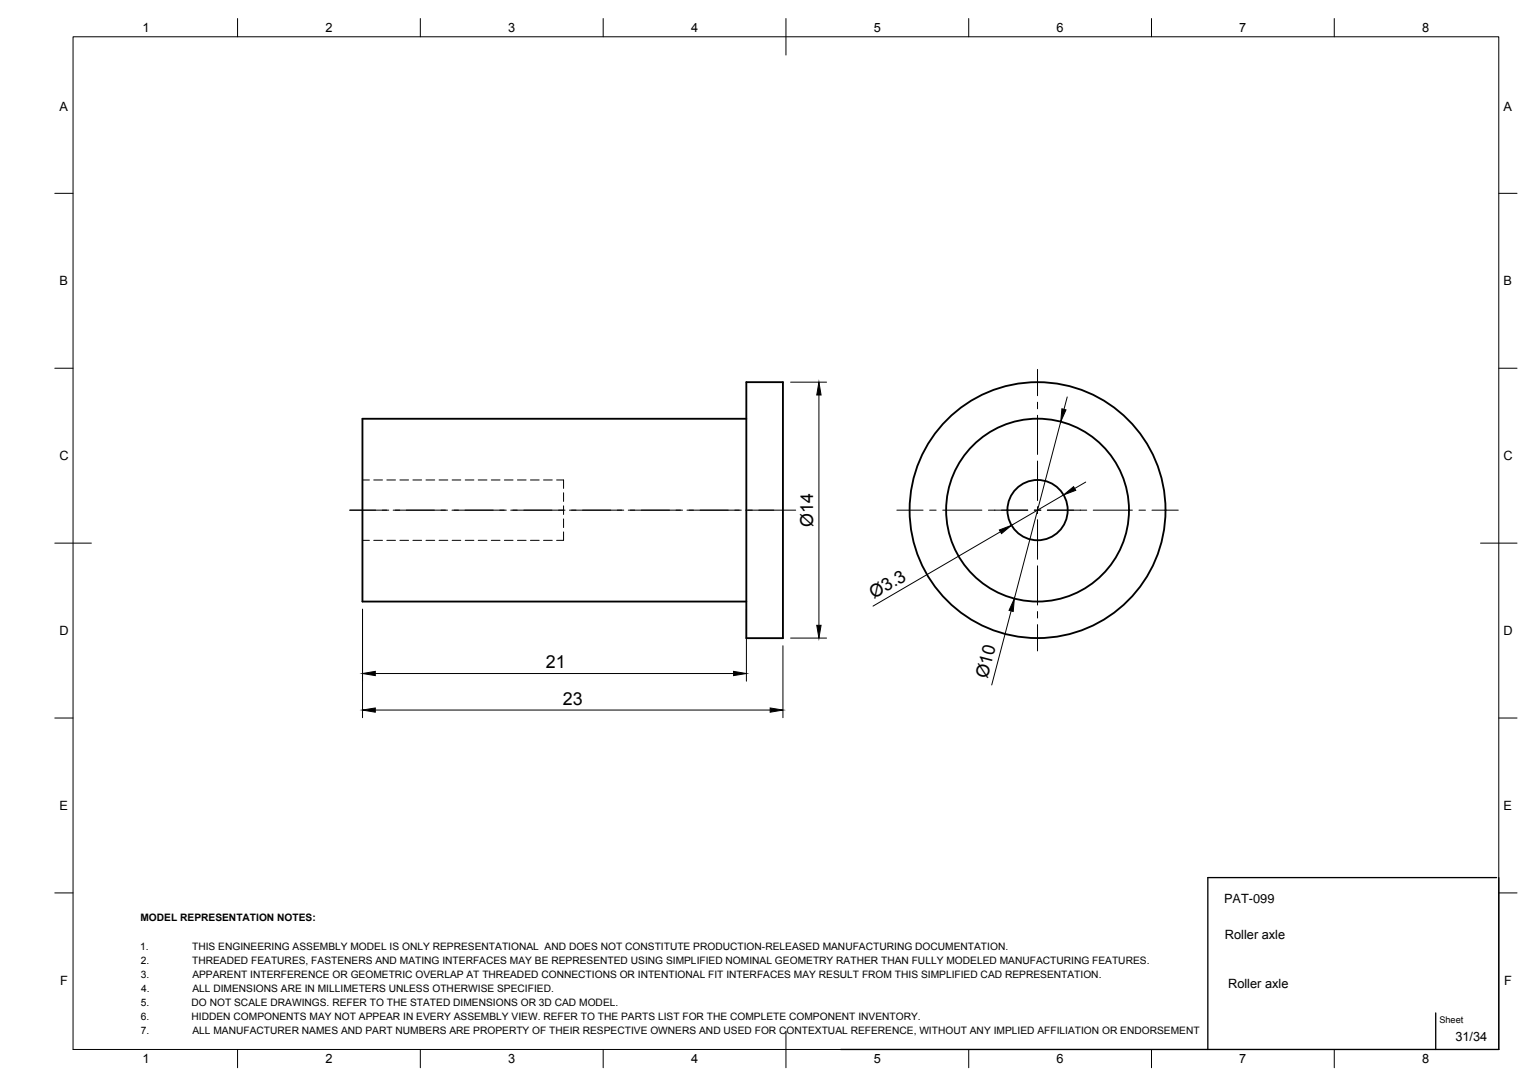
ISO-10303-21;
HEADER;
/* Generated by software containing ST-Developer
 * from STEP Tools, Inc. (www.steptools.com) 
 */

FILE_DESCRIPTION(
/* description */ ('PAT-099'),
/* implementation_level */ '2;1');

FILE_NAME(
/* name */ 'Roller axle.step',
/* time_stamp */ '2026-10-29T17:25:42-07:00',
/* author */ (''),
/* organization */ (''),
/* preprocessor_version */ 'ST-DEVELOPER v20.2',
/* originating_system */ 'Autodesk Translation Framework v15.17.0.0',
/* authorisation */ '');

FILE_SCHEMA (('AUTOMOTIVE_DESIGN { 1 0 10303 214 3 1 1 }'));
ENDSEC;

DATA;
#10=MECHANICAL_DESIGN_GEOMETRIC_PRESENTATION_REPRESENTATION('',(#352),#11035);
#302=SHAPE_REPRESENTATION_RELATIONSHIP('SRR','None',#11173,#327);
#327=ADVANCED_BREP_SHAPE_REPRESENTATION('',(#384),#11023);
#352=STYLED_ITEM('',(#11386),#384);
#384=MANIFOLD_SOLID_BREP('Body1',#4721);
#505=FACE_BOUND('',#1242,.T.);
#506=FACE_BOUND('',#1247,.T.);
#621=PLANE('',#5434);
#622=PLANE('',#5435);
#623=PLANE('',#5440);
#624=PLANE('',#5443);
#854=FACE_OUTER_BOUND('',#1239,.T.);
#855=FACE_OUTER_BOUND('',#1240,.T.);
#856=FACE_OUTER_BOUND('',#1241,.T.);
#857=FACE_OUTER_BOUND('',#1243,.T.);
#858=FACE_OUTER_BOUND('',#1244,.T.);
#859=FACE_OUTER_BOUND('',#1245,.T.);
#860=FACE_OUTER_BOUND('',#1246,.T.);
#1239=EDGE_LOOP('',(#3983,#3984,#3985,#3986));
#1240=EDGE_LOOP('',(#3987));
#1241=EDGE_LOOP('',(#3988));
#1242=EDGE_LOOP('',(#3989));
#1243=EDGE_LOOP('',(#3990,#3991,#3992,#3993));
#1244=EDGE_LOOP('',(#3994));
#1245=EDGE_LOOP('',(#3995,#3996,#3997,#3998));
#1246=EDGE_LOOP('',(#3999));
#1247=EDGE_LOOP('',(#4000));
#1547=LINE('',#10216,#1799);
#1548=LINE('',#10226,#1800);
#1549=LINE('',#10232,#1801);
#1799=VECTOR('',#6706,0.165);
#1800=VECTOR('',#6719,0.7);
#1801=VECTOR('',#6728,0.5);
#2041=CIRCLE('',#5432,0.165);
#2042=CIRCLE('',#5433,0.165);
#2043=CIRCLE('',#5436,0.7);
#2044=CIRCLE('',#5437,0.5);
#2045=CIRCLE('',#5439,0.7);
#2046=CIRCLE('',#5442,0.5);
#2425=VERTEX_POINT('',#10213);
#2426=VERTEX_POINT('',#10215);
#2427=VERTEX_POINT('',#10220);
#2428=VERTEX_POINT('',#10222);
#2429=VERTEX_POINT('',#10225);
#2430=VERTEX_POINT('',#10230);
#2968=EDGE_CURVE('',#2425,#2425,#2041,.T.);
#2969=EDGE_CURVE('',#2425,#2426,#1547,.T.);
#2970=EDGE_CURVE('',#2426,#2426,#2042,.T.);
#2971=EDGE_CURVE('',#2427,#2427,#2043,.T.);
#2972=EDGE_CURVE('',#2428,#2428,#2044,.T.);
#2973=EDGE_CURVE('',#2427,#2429,#1548,.T.);
#2974=EDGE_CURVE('',#2429,#2429,#2045,.T.);
#2975=EDGE_CURVE('',#2430,#2430,#2046,.T.);
#2976=EDGE_CURVE('',#2430,#2428,#1549,.T.);
#3983=ORIENTED_EDGE('',*,*,#2968,.F.);
#3984=ORIENTED_EDGE('',*,*,#2969,.T.);
#3985=ORIENTED_EDGE('',*,*,#2970,.F.);
#3986=ORIENTED_EDGE('',*,*,#2969,.F.);
#3987=ORIENTED_EDGE('',*,*,#2968,.T.);
#3988=ORIENTED_EDGE('',*,*,#2971,.T.);
#3989=ORIENTED_EDGE('',*,*,#2972,.F.);
#3990=ORIENTED_EDGE('',*,*,#2971,.F.);
#3991=ORIENTED_EDGE('',*,*,#2973,.T.);
#3992=ORIENTED_EDGE('',*,*,#2974,.T.);
#3993=ORIENTED_EDGE('',*,*,#2973,.F.);
#3994=ORIENTED_EDGE('',*,*,#2974,.F.);
#3995=ORIENTED_EDGE('',*,*,#2975,.F.);
#3996=ORIENTED_EDGE('',*,*,#2976,.T.);
#3997=ORIENTED_EDGE('',*,*,#2972,.T.);
#3998=ORIENTED_EDGE('',*,*,#2976,.F.);
#3999=ORIENTED_EDGE('',*,*,#2975,.T.);
#4000=ORIENTED_EDGE('',*,*,#2970,.T.);
#4401=CYLINDRICAL_SURFACE('',#5431,0.165);
#4402=CYLINDRICAL_SURFACE('',#5438,0.7);
#4403=CYLINDRICAL_SURFACE('',#5441,0.5);
#4619=ADVANCED_FACE('',(#854),#4401,.F.);
#4620=ADVANCED_FACE('',(#855),#621,.T.);
#4621=ADVANCED_FACE('',(#856,#505),#622,.T.);
#4622=ADVANCED_FACE('',(#857),#4402,.T.);
#4623=ADVANCED_FACE('',(#858),#623,.F.);
#4624=ADVANCED_FACE('',(#859),#4403,.T.);
#4625=ADVANCED_FACE('',(#860,#506),#624,.T.);
#4721=CLOSED_SHELL('',(#4619,#4620,#4621,#4622,#4623,#4624,#4625));
#5430=AXIS2_PLACEMENT_3D('',#10211,#6700,#6701);
#5431=AXIS2_PLACEMENT_3D('',#10212,#6702,#6703);
#5432=AXIS2_PLACEMENT_3D('',#10214,#6704,#6705);
#5433=AXIS2_PLACEMENT_3D('',#10217,#6707,#6708);
#5434=AXIS2_PLACEMENT_3D('',#10218,#6709,#6710);
#5435=AXIS2_PLACEMENT_3D('',#10219,#6711,#6712);
#5436=AXIS2_PLACEMENT_3D('',#10221,#6713,#6714);
#5437=AXIS2_PLACEMENT_3D('',#10223,#6715,#6716);
#5438=AXIS2_PLACEMENT_3D('',#10224,#6717,#6718);
#5439=AXIS2_PLACEMENT_3D('',#10227,#6720,#6721);
#5440=AXIS2_PLACEMENT_3D('',#10228,#6722,#6723);
#5441=AXIS2_PLACEMENT_3D('',#10229,#6724,#6725);
#5442=AXIS2_PLACEMENT_3D('',#10231,#6726,#6727);
#5443=AXIS2_PLACEMENT_3D('',#10233,#6729,#6730);
#6700=DIRECTION('axis',(0.,0.,1.));
#6701=DIRECTION('refdir',(1.,0.,0.));
#6702=DIRECTION('center_axis',(0.,0.,1.));
#6703=DIRECTION('ref_axis',(1.,0.,0.));
#6704=DIRECTION('center_axis',(0.,0.,1.));
#6705=DIRECTION('ref_axis',(1.,0.,0.));
#6706=DIRECTION('',(0.,0.,1.));
#6707=DIRECTION('center_axis',(0.,0.,-1.));
#6708=DIRECTION('ref_axis',(1.,0.,0.));
#6709=DIRECTION('center_axis',(0.,0.,1.));
#6710=DIRECTION('ref_axis',(1.,0.,0.));
#6711=DIRECTION('center_axis',(0.,0.,1.));
#6712=DIRECTION('ref_axis',(1.,0.,0.));
#6713=DIRECTION('center_axis',(0.,0.,1.));
#6714=DIRECTION('ref_axis',(1.,0.,0.));
#6715=DIRECTION('center_axis',(0.,0.,1.));
#6716=DIRECTION('ref_axis',(1.,0.,0.));
#6717=DIRECTION('center_axis',(0.,0.,1.));
#6718=DIRECTION('ref_axis',(1.,0.,0.));
#6719=DIRECTION('',(0.,0.,-1.));
#6720=DIRECTION('center_axis',(0.,0.,1.));
#6721=DIRECTION('ref_axis',(1.,0.,0.));
#6722=DIRECTION('center_axis',(0.,0.,1.));
#6723=DIRECTION('ref_axis',(1.,0.,0.));
#6724=DIRECTION('center_axis',(0.,0.,1.));
#6725=DIRECTION('ref_axis',(1.,0.,0.));
#6726=DIRECTION('center_axis',(0.,0.,1.));
#6727=DIRECTION('ref_axis',(1.,0.,0.));
#6728=DIRECTION('',(0.,0.,-1.));
#6729=DIRECTION('center_axis',(0.,0.,1.));
#6730=DIRECTION('ref_axis',(1.,0.,0.));
#10211=CARTESIAN_POINT('',(0.,0.,0.));
#10212=CARTESIAN_POINT('Origin',(4.,0.,5.2));
#10213=CARTESIAN_POINT('',(3.835,-2.02066721859313E-17,5.2));
#10214=CARTESIAN_POINT('Origin',(4.,0.,5.2));
#10215=CARTESIAN_POINT('',(3.835,2.02066721859313E-17,6.3));
#10216=CARTESIAN_POINT('',(3.835,-2.02066721859313E-17,5.2));
#10217=CARTESIAN_POINT('Origin',(4.,0.,6.3));
#10218=CARTESIAN_POINT('Origin',(4.,0.,5.2));
#10219=CARTESIAN_POINT('Origin',(4.,0.,4.2));
#10220=CARTESIAN_POINT('',(3.3,-8.57252759403147E-17,4.2));
#10221=CARTESIAN_POINT('Origin',(4.,0.,4.2));
#10222=CARTESIAN_POINT('',(3.5,-6.12323399573677E-17,4.2));
#10223=CARTESIAN_POINT('Origin',(4.,0.,4.2));
#10224=CARTESIAN_POINT('Origin',(4.,0.,4.));
#10225=CARTESIAN_POINT('',(3.3,-8.57252759403147E-17,4.));
#10226=CARTESIAN_POINT('',(3.3,-8.57252759403147E-17,4.));
#10227=CARTESIAN_POINT('Origin',(4.,0.,4.));
#10228=CARTESIAN_POINT('Origin',(4.,0.,4.));
#10229=CARTESIAN_POINT('Origin',(4.,0.,4.2));
#10230=CARTESIAN_POINT('',(3.5,-6.12323399573677E-17,6.3));
#10231=CARTESIAN_POINT('Origin',(4.,0.,6.3));
#10232=CARTESIAN_POINT('',(3.5,-6.12323399573677E-17,4.2));
#10233=CARTESIAN_POINT('Origin',(4.,0.,6.3));
#10990=UNCERTAINTY_MEASURE_WITH_UNIT(LENGTH_MEASURE(0.001),#11036,
'DISTANCE_ACCURACY_VALUE',
'Maximum model space distance between geometric entities at asserted c
onnectivities');
#11002=UNCERTAINTY_MEASURE_WITH_UNIT(LENGTH_MEASURE(0.001),#11036,
'DISTANCE_ACCURACY_VALUE',
'Maximum model space distance between geometric entities at asserted c
onnectivities');
#11023=(
GEOMETRIC_REPRESENTATION_CONTEXT(3)
GLOBAL_UNCERTAINTY_ASSIGNED_CONTEXT((#10990))
GLOBAL_UNIT_ASSIGNED_CONTEXT((#11036,#11038,#11039))
REPRESENTATION_CONTEXT('','3D')
);
#11035=(
GEOMETRIC_REPRESENTATION_CONTEXT(3)
GLOBAL_UNCERTAINTY_ASSIGNED_CONTEXT((#11002))
GLOBAL_UNIT_ASSIGNED_CONTEXT((#11036,#11038,#11039))
REPRESENTATION_CONTEXT('','3D')
);
#11036=(
LENGTH_UNIT()
NAMED_UNIT(*)
SI_UNIT(.CENTI.,.METRE.)
);
#11038=(
NAMED_UNIT(*)
PLANE_ANGLE_UNIT()
SI_UNIT($,.RADIAN.)
);
#11039=(
NAMED_UNIT(*)
SI_UNIT($,.STERADIAN.)
SOLID_ANGLE_UNIT()
);
#11060=SHAPE_DEFINITION_REPRESENTATION(#11098,#11173);
#11098=PRODUCT_DEFINITION_SHAPE('',$,#11206);
#11173=SHAPE_REPRESENTATION('',(#5430),#11023);
#11185=PRODUCT_DEFINITION_CONTEXT('part definition',#11283,'design');
#11206=PRODUCT_DEFINITION('Roller axle','Roller axle',#11238,#11185);
#11238=PRODUCT_DEFINITION_FORMATION('',$,#11305);
#11283=APPLICATION_CONTEXT(
'Core Data for Automotive Mechanical Design Process');
#11284=PRODUCT_CONTEXT('part definition',#11283,'mechanical');
#11305=PRODUCT('Roller axle','Roller axle','Roller axle',(#11284));
#11380=COLOUR_RGB('Grey',0.48,0.52,0.57);
#11381=FILL_AREA_STYLE_COLOUR('',#11380);
#11382=FILL_AREA_STYLE('',(#11381));
#11383=SURFACE_STYLE_FILL_AREA(#11382);
#11384=SURFACE_SIDE_STYLE('',(#11383));
#11385=SURFACE_STYLE_USAGE(.BOTH.,#11384);
#11386=PRESENTATION_STYLE_ASSIGNMENT((#11385));
ENDSEC;
END-ISO-10303-21;
